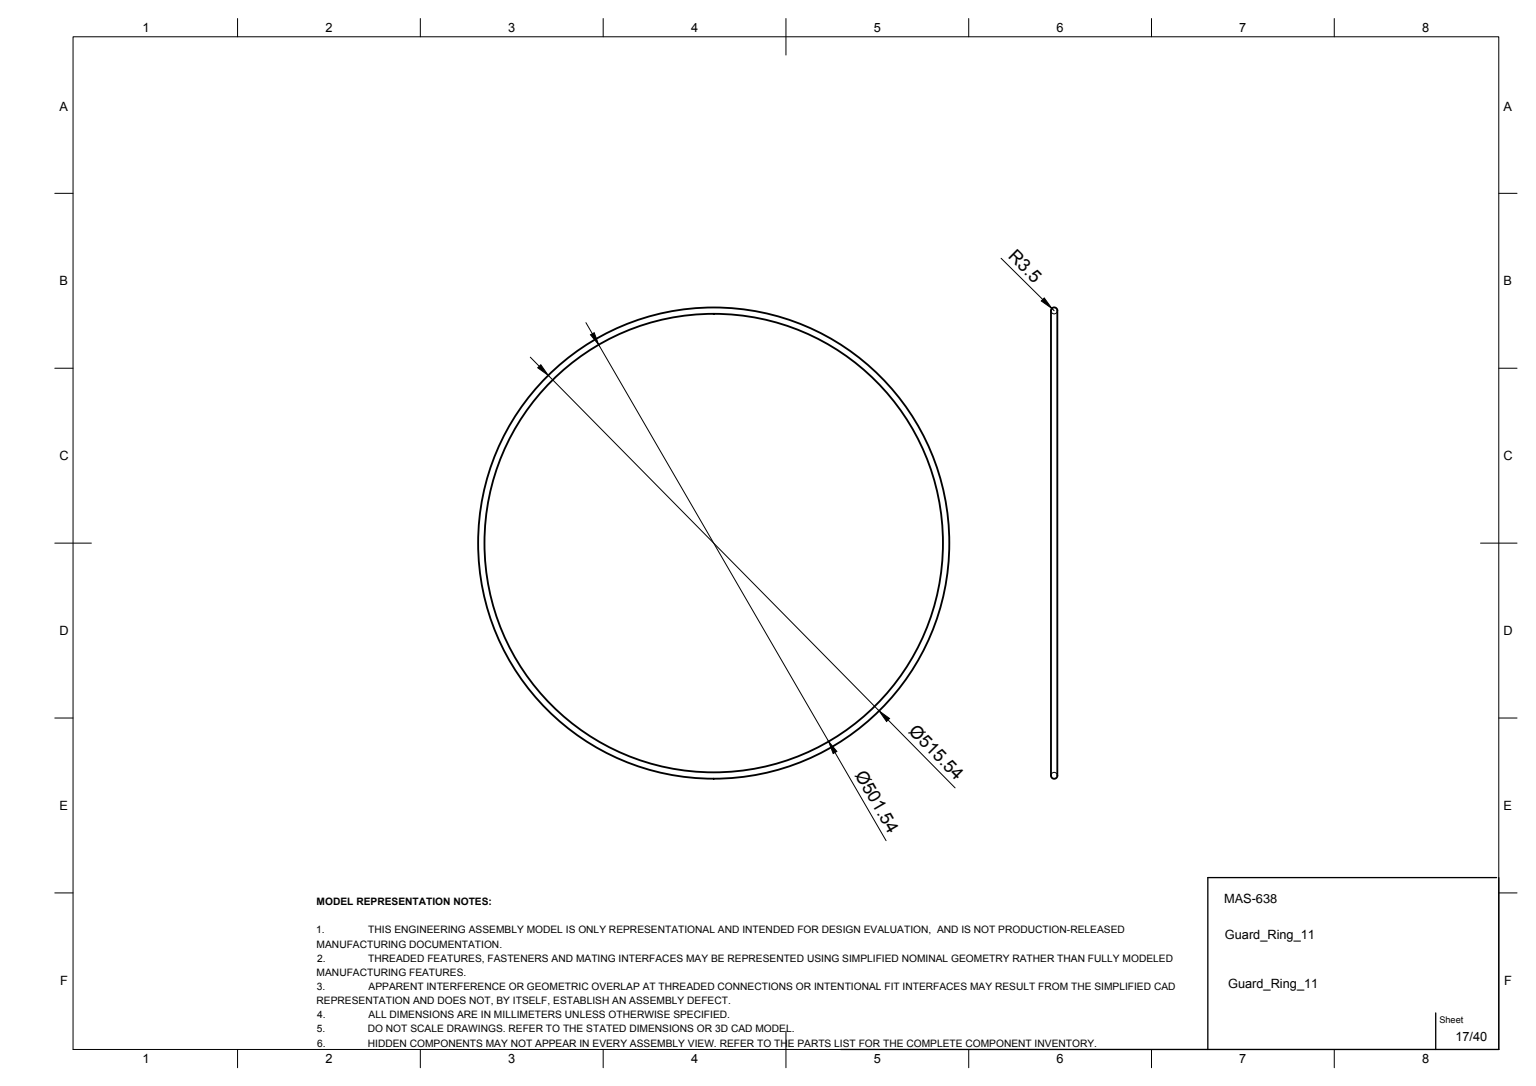
ISO-10303-21;
HEADER;
FILE_DESCRIPTION((''),'2;1');
FILE_NAME('Guard_Ring_11.step','2026-10-09T12:00:21-07:00',(''),(''),'','','');
FILE_SCHEMA (('AUTOMOTIVE_DESIGN { 1 0 10303 214 3 1 1 }'));
ENDSEC;
DATA;
#10=MECHANICAL_DESIGN_GEOMETRIC_PRESENTATION_REPRESENTATION('',(#411,#412),#10334);
#344=SHAPE_REPRESENTATION_RELATIONSHIP('SRR','None',#10460,#376) ;
#376=ADVANCED_BREP_SHAPE_REPRESENTATION('',(#448),#10312) ;
#411=STYLED_ITEM('',(#10631),#3377) ;
#412=STYLED_ITEM('',(#10632),#448) ;
#448=MANIFOLD_SOLID_BREP('Body1',#3570) ;
#869=FACE_OUTER_BOUND('',#1069,.T.) ;
#1069=EDGE_LOOP('',(#2389,#2390,#2391,#2392)) ;
#1296=CIRCLE('',#4015,0.349999999999999) ;
#1297=CIRCLE('',#4016,25.0768144613668) ;
#1523=VERTEX_POINT('',#5703) ;
#1851=EDGE_CURVE('',#1523,#1523,#1296,.T.) ;
#1852=EDGE_CURVE('',#1523,#1523,#1297,.T.) ;
#2389=ORIENTED_EDGE('',*,*,#1851,.F.) ;
#2390=ORIENTED_EDGE('',*,*,#1852,.T.) ;
#2391=ORIENTED_EDGE('',*,*,#1851,.T.) ;
#2392=ORIENTED_EDGE('',*,*,#1852,.F.) ;
#3315=TOROIDAL_SURFACE('',#4014,25.4268144613668,0.349999999999999) ;
#3377=ADVANCED_FACE('',(#869),#3315,.T.) ;
#3570=CLOSED_SHELL('',(#3377)) ;
#4013=AXIS2_PLACEMENT_3D('',#5701,#4587,#4588) ;
#4014=AXIS2_PLACEMENT_3D('',#5702,#4589,#4590) ;
#4015=AXIS2_PLACEMENT_3D('',#5704,#4591,#4592) ;
#4016=AXIS2_PLACEMENT_3D('',#5705,#4593,#4594) ;
#4587=DIRECTION('axis',(0.,0.,1.)) ;
#4588=DIRECTION('refdir',(1.,0.,0.)) ;
#4589=DIRECTION('center_axis',(-6.42891162084177E-17,-1.,-1.01883556321148E-16)) ;
#4590=DIRECTION('ref_axis',(1.,0.,0.)) ;
#4591=DIRECTION('center_axis',(0.,1.01883556321148E-16,-1.)) ;
#4592=DIRECTION('ref_axis',(-1.,0.,0.)) ;
#4593=DIRECTION('center_axis',(6.42891162084177E-17,1.,1.01883556321148E-16)) ;
#4594=DIRECTION('ref_axis',(1.,-6.42891162084177E-17,-6.55000379205715E-33)) ;
#5701=CARTESIAN_POINT('',(0.,0.,0.)) ;
#5702=CARTESIAN_POINT('Origin',(23.47768801576,67.3831179463143,68.2224337400009)) ;
#5703=CARTESIAN_POINT('',(-1.5991264456068,67.3831179463143,68.2224337400009)) ;
#5704=CARTESIAN_POINT('Origin',(-1.9491264456068,67.3831179463143,68.2224337400009)) ;
#5705=CARTESIAN_POINT('Origin',(23.47768801576,67.3831179463143,68.2224337400009)) ;
#10275=UNCERTAINTY_MEASURE_WITH_UNIT(LENGTH_MEASURE(0.001),#10335,
'DISTANCE_ACCURACY_VALUE',
'Maximum model space distance between geometric entities at asserted c
onnectivities') ;
#10297=UNCERTAINTY_MEASURE_WITH_UNIT(LENGTH_MEASURE(0.001),#10335,
'DISTANCE_ACCURACY_VALUE',
'Maximum model space distance between geometric entities at asserted c
onnectivities') ;
#10312=(
GEOMETRIC_REPRESENTATION_CONTEXT(3)
GLOBAL_UNCERTAINTY_ASSIGNED_CONTEXT((#10275))
GLOBAL_UNIT_ASSIGNED_CONTEXT((#10335,#10337,#10338))
REPRESENTATION_CONTEXT('','3D')
) ;
#10334=(
GEOMETRIC_REPRESENTATION_CONTEXT(3)
GLOBAL_UNCERTAINTY_ASSIGNED_CONTEXT((#10297))
GLOBAL_UNIT_ASSIGNED_CONTEXT((#10335,#10337,#10338))
REPRESENTATION_CONTEXT('','3D')
) ;
#10335=(
LENGTH_UNIT()
NAMED_UNIT(*)
SI_UNIT(.CENTI.,.METRE.)
) ;
#10337=(
NAMED_UNIT(*)
PLANE_ANGLE_UNIT()
SI_UNIT($,.RADIAN.)
) ;
#10338=(
NAMED_UNIT(*)
SI_UNIT($,.STERADIAN.)
SOLID_ANGLE_UNIT()
) ;
#10353=SHAPE_DEFINITION_REPRESENTATION(#10389,#10460) ;
#10389=PRODUCT_DEFINITION_SHAPE('',$,#10497) ;
#10460=SHAPE_REPRESENTATION('',(#4013),#10312) ;
#10482=PRODUCT_DEFINITION_CONTEXT('part definition',#10592,'design') ;
#10497=PRODUCT_DEFINITION('Guard_Ring_11','Guard_Ring_11',#10533,#10482) ;
#10533=PRODUCT_DEFINITION_FORMATION('',$,#10608) ;
#10592=APPLICATION_CONTEXT(
'Core Data for Automotive Mechanical Design Process') ;
#10593=PRODUCT_CONTEXT('part definition',#10592,'mechanical') ;
#10608=PRODUCT('Guard_Ring_11','Guard_Ring_11',$,(#10593)) ;
#10631=PRESENTATION_STYLE_ASSIGNMENT((#10635)) ;
#10632=PRESENTATION_STYLE_ASSIGNMENT((#10636)) ;
#10635=SURFACE_STYLE_USAGE(.BOTH.,#10639) ;
#10636=SURFACE_STYLE_USAGE(.BOTH.,#10640) ;
#10639=SURFACE_SIDE_STYLE('',(#10643)) ;
#10640=SURFACE_SIDE_STYLE('',(#10644)) ;
#10643=SURFACE_STYLE_FILL_AREA(#10647) ;
#10644=SURFACE_STYLE_FILL_AREA(#10648) ;
#10647=FILL_AREA_STYLE('Opaque(25,25,25)',(#10651)) ;
#10648=FILL_AREA_STYLE('Opaque(202,209,238)',(#10652)) ;
#10651=FILL_AREA_STYLE_COLOUR('Opaque(25,25,25)',#10655) ;
#10652=FILL_AREA_STYLE_COLOUR('Opaque(202,209,238)',#10656) ;
#10655=COLOUR_RGB('Opaque(25,25,25)', 0.09019608, 0.27058824, 0.51372549) ;
#10656=COLOUR_RGB('Opaque(202,209,238)', 0.40784314, 0.44705882, 0.49803922) ;
ENDSEC;
END-ISO-10303-21;
